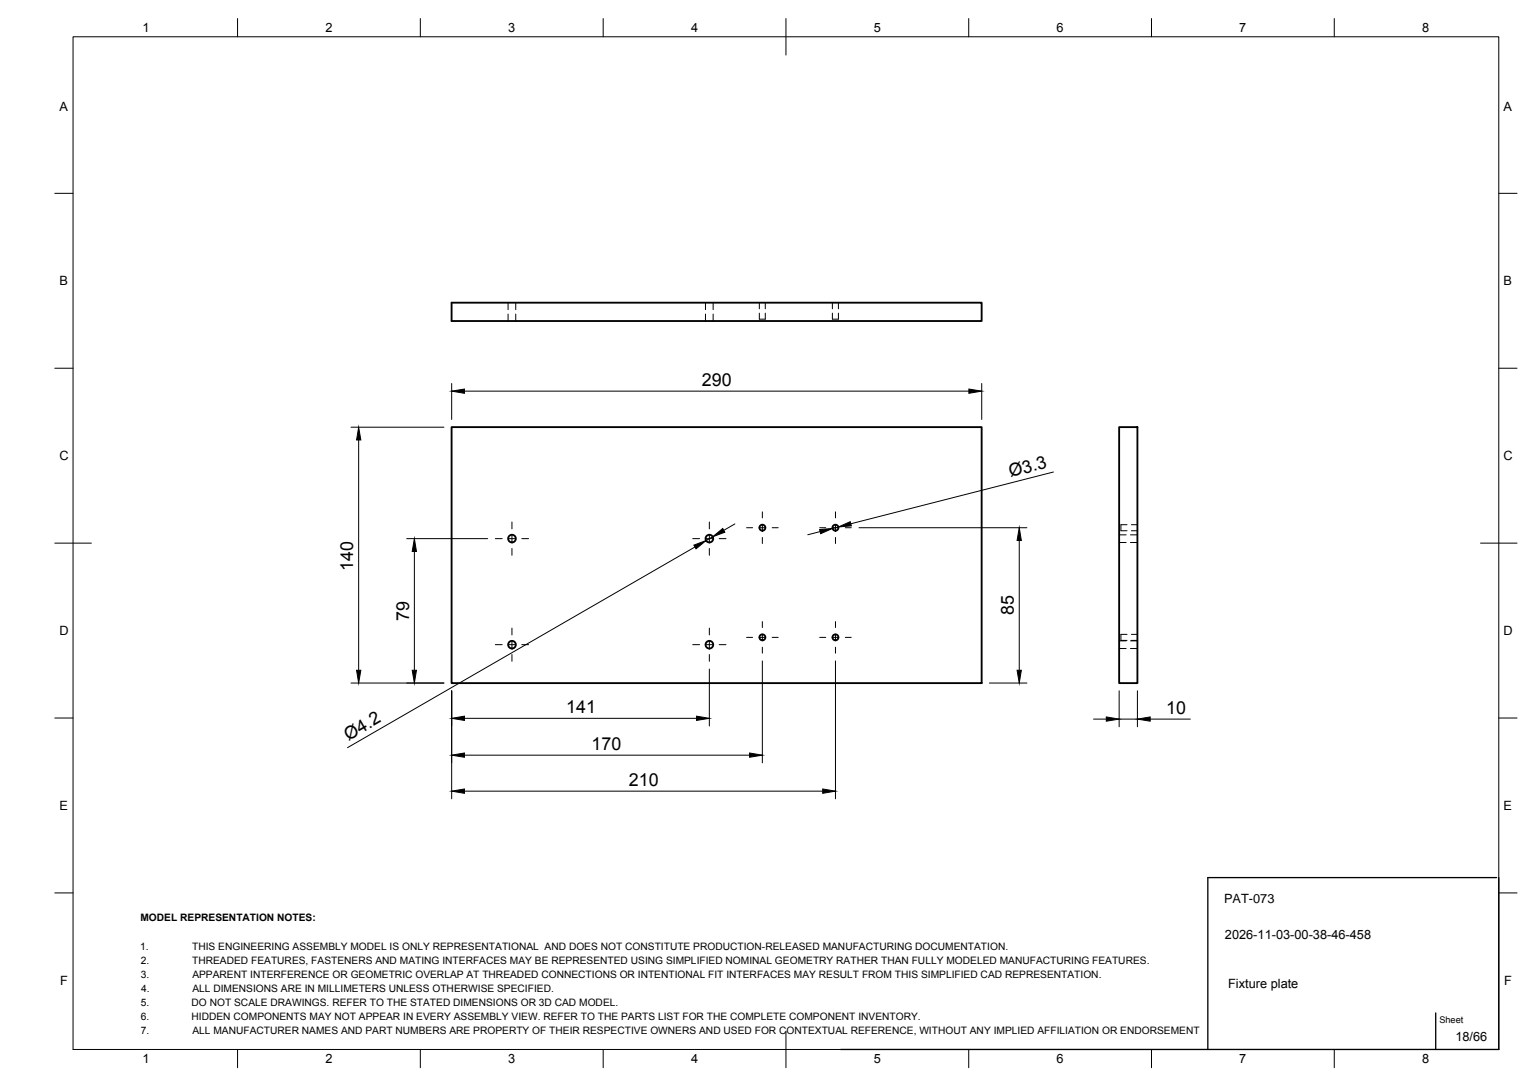
ISO-10303-21;
HEADER;
/* Generated by software containing ST-Developer
 * from STEP Tools, Inc. (www.steptools.com) 
 */

FILE_DESCRIPTION(
/* description */ ('Manual piston pump'),
/* implementation_level */ '2;1');

FILE_NAME(
/* name */ 'Fixture plate.step',
/* time_stamp */ '2026-11-02T16:54:23-08:00',
/* author */ (''),
/* organization */ (''),
/* preprocessor_version */ 'ST-DEVELOPER v20.2',
/* originating_system */ 'Autodesk Translation Framework v15.17.0.0',
/* authorisation */ '');

FILE_SCHEMA (('AUTOMOTIVE_DESIGN { 1 0 10303 214 3 1 1 }'));
ENDSEC;

DATA;
#10=MECHANICAL_DESIGN_GEOMETRIC_PRESENTATION_REPRESENTATION('',(#704),#19043);
#578=SHAPE_REPRESENTATION_RELATIONSHIP('SRR','None',#19324,#641);
#641=ADVANCED_BREP_SHAPE_REPRESENTATION('',(#775),#18991);
#704=STYLED_ITEM('',(#19661),#775);
#775=MANIFOLD_SOLID_BREP('Body1',#9489);
#889=FACE_BOUND('',#2092,.T.);
#890=FACE_BOUND('',#2093,.T.);
#891=FACE_BOUND('',#2094,.T.);
#892=FACE_BOUND('',#2095,.T.);
#893=FACE_BOUND('',#2096,.T.);
#894=FACE_BOUND('',#2097,.T.);
#895=FACE_BOUND('',#2098,.T.);
#896=FACE_BOUND('',#2099,.T.);
#897=FACE_BOUND('',#2101,.T.);
#898=FACE_BOUND('',#2102,.T.);
#899=FACE_BOUND('',#2103,.T.);
#900=FACE_BOUND('',#2104,.T.);
#1147=CYLINDRICAL_SURFACE('',#10531,0.165);
#1148=CYLINDRICAL_SURFACE('',#10535,0.165);
#1149=CYLINDRICAL_SURFACE('',#10539,0.165);
#1150=CYLINDRICAL_SURFACE('',#10543,0.165);
#1151=CYLINDRICAL_SURFACE('',#10547,0.21);
#1152=CYLINDRICAL_SURFACE('',#10550,0.21);
#1153=CYLINDRICAL_SURFACE('',#10553,0.21);
#1154=CYLINDRICAL_SURFACE('',#10556,0.21);
#1438=FACE_OUTER_BOUND('',#2075,.T.);
#1439=FACE_OUTER_BOUND('',#2076,.T.);
#1440=FACE_OUTER_BOUND('',#2077,.T.);
#1441=FACE_OUTER_BOUND('',#2078,.T.);
#1442=FACE_OUTER_BOUND('',#2079,.T.);
#1443=FACE_OUTER_BOUND('',#2080,.T.);
#1444=FACE_OUTER_BOUND('',#2081,.T.);
#1445=FACE_OUTER_BOUND('',#2082,.T.);
#1446=FACE_OUTER_BOUND('',#2083,.T.);
#1447=FACE_OUTER_BOUND('',#2084,.T.);
#1448=FACE_OUTER_BOUND('',#2085,.T.);
#1449=FACE_OUTER_BOUND('',#2086,.T.);
#1450=FACE_OUTER_BOUND('',#2087,.T.);
#1451=FACE_OUTER_BOUND('',#2088,.T.);
#1452=FACE_OUTER_BOUND('',#2089,.T.);
#1453=FACE_OUTER_BOUND('',#2090,.T.);
#1454=FACE_OUTER_BOUND('',#2091,.T.);
#1455=FACE_OUTER_BOUND('',#2100,.T.);
#2075=EDGE_LOOP('',(#6865,#6866,#6867,#6868));
#2076=EDGE_LOOP('',(#6869));
#2077=EDGE_LOOP('',(#6870,#6871,#6872,#6873));
#2078=EDGE_LOOP('',(#6874));
#2079=EDGE_LOOP('',(#6875,#6876,#6877,#6878));
#2080=EDGE_LOOP('',(#6879));
#2081=EDGE_LOOP('',(#6880,#6881,#6882,#6883));
#2082=EDGE_LOOP('',(#6884));
#2083=EDGE_LOOP('',(#6885,#6886,#6887,#6888));
#2084=EDGE_LOOP('',(#6889,#6890,#6891,#6892));
#2085=EDGE_LOOP('',(#6893,#6894,#6895,#6896));
#2086=EDGE_LOOP('',(#6897,#6898,#6899,#6900));
#2087=EDGE_LOOP('',(#6901,#6902,#6903,#6904));
#2088=EDGE_LOOP('',(#6905,#6906,#6907,#6908));
#2089=EDGE_LOOP('',(#6909,#6910,#6911,#6912));
#2090=EDGE_LOOP('',(#6913,#6914,#6915,#6916));
#2091=EDGE_LOOP('',(#6917,#6918,#6919,#6920));
#2092=EDGE_LOOP('',(#6921));
#2093=EDGE_LOOP('',(#6922));
#2094=EDGE_LOOP('',(#6923));
#2095=EDGE_LOOP('',(#6924));
#2096=EDGE_LOOP('',(#6925));
#2097=EDGE_LOOP('',(#6926));
#2098=EDGE_LOOP('',(#6927));
#2099=EDGE_LOOP('',(#6928));
#2100=EDGE_LOOP('',(#6929,#6930,#6931,#6932));
#2101=EDGE_LOOP('',(#6933));
#2102=EDGE_LOOP('',(#6934));
#2103=EDGE_LOOP('',(#6935));
#2104=EDGE_LOOP('',(#6936));
#2786=CIRCLE('',#10532,0.165);
#2787=CIRCLE('',#10533,0.165);
#2788=CIRCLE('',#10536,0.165);
#2789=CIRCLE('',#10537,0.165);
#2790=CIRCLE('',#10540,0.165);
#2791=CIRCLE('',#10541,0.165);
#2792=CIRCLE('',#10544,0.165);
#2793=CIRCLE('',#10545,0.165);
#2794=CIRCLE('',#10548,0.21);
#2795=CIRCLE('',#10549,0.21);
#2796=CIRCLE('',#10551,0.21);
#2797=CIRCLE('',#10552,0.21);
#2798=CIRCLE('',#10554,0.21);
#2799=CIRCLE('',#10555,0.21);
#2800=CIRCLE('',#10557,0.21);
#2801=CIRCLE('',#10558,0.21);
#3305=LINE('',#15337,#3909);
#3306=LINE('',#15344,#3910);
#3307=LINE('',#15351,#3911);
#3308=LINE('',#15358,#3912);
#3309=LINE('',#15365,#3913);
#3310=LINE('',#15371,#3914);
#3311=LINE('',#15377,#3915);
#3312=LINE('',#15383,#3916);
#3313=LINE('',#15388,#3917);
#3314=LINE('',#15390,#3918);
#3315=LINE('',#15392,#3919);
#3316=LINE('',#15393,#3920);
#3317=LINE('',#15396,#3921);
#3318=LINE('',#15398,#3922);
#3319=LINE('',#15399,#3923);
#3320=LINE('',#15402,#3924);
#3321=LINE('',#15404,#3925);
#3322=LINE('',#15405,#3926);
#3323=LINE('',#15407,#3927);
#3324=LINE('',#15408,#3928);
#3909=VECTOR('',#12233,0.165);
#3910=VECTOR('',#12242,0.165);
#3911=VECTOR('',#12251,0.165);
#3912=VECTOR('',#12260,0.165);
#3913=VECTOR('',#12269,0.21);
#3914=VECTOR('',#12276,0.21);
#3915=VECTOR('',#12283,0.21);
#3916=VECTOR('',#12290,0.21);
#3917=VECTOR('',#12295,1.);
#3918=VECTOR('',#12296,1.);
#3919=VECTOR('',#12297,1.);
#3920=VECTOR('',#12298,1.);
#3921=VECTOR('',#12301,1.);
#3922=VECTOR('',#12302,1.);
#3923=VECTOR('',#12303,1.);
#3924=VECTOR('',#12306,1.);
#3925=VECTOR('',#12307,1.);
#3926=VECTOR('',#12308,1.);
#3927=VECTOR('',#12311,1.);
#3928=VECTOR('',#12312,1.);
#4549=VERTEX_POINT('',#15334);
#4550=VERTEX_POINT('',#15336);
#4551=VERTEX_POINT('',#15341);
#4552=VERTEX_POINT('',#15343);
#4553=VERTEX_POINT('',#15348);
#4554=VERTEX_POINT('',#15350);
#4555=VERTEX_POINT('',#15355);
#4556=VERTEX_POINT('',#15357);
#4557=VERTEX_POINT('',#15362);
#4558=VERTEX_POINT('',#15364);
#4559=VERTEX_POINT('',#15368);
#4560=VERTEX_POINT('',#15370);
#4561=VERTEX_POINT('',#15374);
#4562=VERTEX_POINT('',#15376);
#4563=VERTEX_POINT('',#15380);
#4564=VERTEX_POINT('',#15382);
#4565=VERTEX_POINT('',#15386);
#4566=VERTEX_POINT('',#15387);
#4567=VERTEX_POINT('',#15389);
#4568=VERTEX_POINT('',#15391);
#4569=VERTEX_POINT('',#15395);
#4570=VERTEX_POINT('',#15397);
#4571=VERTEX_POINT('',#15401);
#4572=VERTEX_POINT('',#15403);
#5419=EDGE_CURVE('',#4549,#4549,#2786,.T.);
#5420=EDGE_CURVE('',#4549,#4550,#3305,.T.);
#5421=EDGE_CURVE('',#4550,#4550,#2787,.T.);
#5422=EDGE_CURVE('',#4551,#4551,#2788,.T.);
#5423=EDGE_CURVE('',#4551,#4552,#3306,.T.);
#5424=EDGE_CURVE('',#4552,#4552,#2789,.T.);
#5425=EDGE_CURVE('',#4553,#4553,#2790,.T.);
#5426=EDGE_CURVE('',#4553,#4554,#3307,.T.);
#5427=EDGE_CURVE('',#4554,#4554,#2791,.T.);
#5428=EDGE_CURVE('',#4555,#4555,#2792,.T.);
#5429=EDGE_CURVE('',#4555,#4556,#3308,.T.);
#5430=EDGE_CURVE('',#4556,#4556,#2793,.T.);
#5431=EDGE_CURVE('',#4557,#4557,#2794,.T.);
#5432=EDGE_CURVE('',#4557,#4558,#3309,.T.);
#5433=EDGE_CURVE('',#4558,#4558,#2795,.T.);
#5434=EDGE_CURVE('',#4559,#4559,#2796,.T.);
#5435=EDGE_CURVE('',#4559,#4560,#3310,.T.);
#5436=EDGE_CURVE('',#4560,#4560,#2797,.T.);
#5437=EDGE_CURVE('',#4561,#4561,#2798,.T.);
#5438=EDGE_CURVE('',#4561,#4562,#3311,.T.);
#5439=EDGE_CURVE('',#4562,#4562,#2799,.T.);
#5440=EDGE_CURVE('',#4563,#4563,#2800,.T.);
#5441=EDGE_CURVE('',#4563,#4564,#3312,.T.);
#5442=EDGE_CURVE('',#4564,#4564,#2801,.T.);
#5443=EDGE_CURVE('',#4565,#4566,#3313,.T.);
#5444=EDGE_CURVE('',#4566,#4567,#3314,.T.);
#5445=EDGE_CURVE('',#4568,#4567,#3315,.T.);
#5446=EDGE_CURVE('',#4565,#4568,#3316,.T.);
#5447=EDGE_CURVE('',#4569,#4565,#3317,.T.);
#5448=EDGE_CURVE('',#4570,#4568,#3318,.T.);
#5449=EDGE_CURVE('',#4569,#4570,#3319,.T.);
#5450=EDGE_CURVE('',#4571,#4569,#3320,.T.);
#5451=EDGE_CURVE('',#4572,#4570,#3321,.T.);
#5452=EDGE_CURVE('',#4571,#4572,#3322,.T.);
#5453=EDGE_CURVE('',#4566,#4571,#3323,.T.);
#5454=EDGE_CURVE('',#4567,#4572,#3324,.T.);
#6865=ORIENTED_EDGE('',*,*,#5419,.F.);
#6866=ORIENTED_EDGE('',*,*,#5420,.T.);
#6867=ORIENTED_EDGE('',*,*,#5421,.F.);
#6868=ORIENTED_EDGE('',*,*,#5420,.F.);
#6869=ORIENTED_EDGE('',*,*,#5419,.T.);
#6870=ORIENTED_EDGE('',*,*,#5422,.F.);
#6871=ORIENTED_EDGE('',*,*,#5423,.T.);
#6872=ORIENTED_EDGE('',*,*,#5424,.F.);
#6873=ORIENTED_EDGE('',*,*,#5423,.F.);
#6874=ORIENTED_EDGE('',*,*,#5422,.T.);
#6875=ORIENTED_EDGE('',*,*,#5425,.F.);
#6876=ORIENTED_EDGE('',*,*,#5426,.T.);
#6877=ORIENTED_EDGE('',*,*,#5427,.F.);
#6878=ORIENTED_EDGE('',*,*,#5426,.F.);
#6879=ORIENTED_EDGE('',*,*,#5425,.T.);
#6880=ORIENTED_EDGE('',*,*,#5428,.F.);
#6881=ORIENTED_EDGE('',*,*,#5429,.T.);
#6882=ORIENTED_EDGE('',*,*,#5430,.F.);
#6883=ORIENTED_EDGE('',*,*,#5429,.F.);
#6884=ORIENTED_EDGE('',*,*,#5428,.T.);
#6885=ORIENTED_EDGE('',*,*,#5431,.F.);
#6886=ORIENTED_EDGE('',*,*,#5432,.T.);
#6887=ORIENTED_EDGE('',*,*,#5433,.F.);
#6888=ORIENTED_EDGE('',*,*,#5432,.F.);
#6889=ORIENTED_EDGE('',*,*,#5434,.F.);
#6890=ORIENTED_EDGE('',*,*,#5435,.T.);
#6891=ORIENTED_EDGE('',*,*,#5436,.F.);
#6892=ORIENTED_EDGE('',*,*,#5435,.F.);
#6893=ORIENTED_EDGE('',*,*,#5437,.F.);
#6894=ORIENTED_EDGE('',*,*,#5438,.T.);
#6895=ORIENTED_EDGE('',*,*,#5439,.F.);
#6896=ORIENTED_EDGE('',*,*,#5438,.F.);
#6897=ORIENTED_EDGE('',*,*,#5440,.F.);
#6898=ORIENTED_EDGE('',*,*,#5441,.T.);
#6899=ORIENTED_EDGE('',*,*,#5442,.F.);
#6900=ORIENTED_EDGE('',*,*,#5441,.F.);
#6901=ORIENTED_EDGE('',*,*,#5443,.T.);
#6902=ORIENTED_EDGE('',*,*,#5444,.T.);
#6903=ORIENTED_EDGE('',*,*,#5445,.F.);
#6904=ORIENTED_EDGE('',*,*,#5446,.F.);
#6905=ORIENTED_EDGE('',*,*,#5447,.T.);
#6906=ORIENTED_EDGE('',*,*,#5446,.T.);
#6907=ORIENTED_EDGE('',*,*,#5448,.F.);
#6908=ORIENTED_EDGE('',*,*,#5449,.F.);
#6909=ORIENTED_EDGE('',*,*,#5450,.T.);
#6910=ORIENTED_EDGE('',*,*,#5449,.T.);
#6911=ORIENTED_EDGE('',*,*,#5451,.F.);
#6912=ORIENTED_EDGE('',*,*,#5452,.F.);
#6913=ORIENTED_EDGE('',*,*,#5453,.T.);
#6914=ORIENTED_EDGE('',*,*,#5452,.T.);
#6915=ORIENTED_EDGE('',*,*,#5454,.F.);
#6916=ORIENTED_EDGE('',*,*,#5444,.F.);
#6917=ORIENTED_EDGE('',*,*,#5454,.T.);
#6918=ORIENTED_EDGE('',*,*,#5451,.T.);
#6919=ORIENTED_EDGE('',*,*,#5448,.T.);
#6920=ORIENTED_EDGE('',*,*,#5445,.T.);
#6921=ORIENTED_EDGE('',*,*,#5442,.T.);
#6922=ORIENTED_EDGE('',*,*,#5439,.T.);
#6923=ORIENTED_EDGE('',*,*,#5436,.T.);
#6924=ORIENTED_EDGE('',*,*,#5433,.T.);
#6925=ORIENTED_EDGE('',*,*,#5430,.T.);
#6926=ORIENTED_EDGE('',*,*,#5427,.T.);
#6927=ORIENTED_EDGE('',*,*,#5424,.T.);
#6928=ORIENTED_EDGE('',*,*,#5421,.T.);
#6929=ORIENTED_EDGE('',*,*,#5453,.F.);
#6930=ORIENTED_EDGE('',*,*,#5443,.F.);
#6931=ORIENTED_EDGE('',*,*,#5447,.F.);
#6932=ORIENTED_EDGE('',*,*,#5450,.F.);
#6933=ORIENTED_EDGE('',*,*,#5431,.T.);
#6934=ORIENTED_EDGE('',*,*,#5434,.T.);
#6935=ORIENTED_EDGE('',*,*,#5437,.T.);
#6936=ORIENTED_EDGE('',*,*,#5440,.T.);
#8655=PLANE('',#10534);
#8656=PLANE('',#10538);
#8657=PLANE('',#10542);
#8658=PLANE('',#10546);
#8659=PLANE('',#10559);
#8660=PLANE('',#10560);
#8661=PLANE('',#10561);
#8662=PLANE('',#10562);
#8663=PLANE('',#10563);
#8664=PLANE('',#10564);
#9043=ADVANCED_FACE('',(#1438),#1147,.F.);
#9044=ADVANCED_FACE('',(#1439),#8655,.T.);
#9045=ADVANCED_FACE('',(#1440),#1148,.F.);
#9046=ADVANCED_FACE('',(#1441),#8656,.T.);
#9047=ADVANCED_FACE('',(#1442),#1149,.F.);
#9048=ADVANCED_FACE('',(#1443),#8657,.T.);
#9049=ADVANCED_FACE('',(#1444),#1150,.F.);
#9050=ADVANCED_FACE('',(#1445),#8658,.T.);
#9051=ADVANCED_FACE('',(#1446),#1151,.F.);
#9052=ADVANCED_FACE('',(#1447),#1152,.F.);
#9053=ADVANCED_FACE('',(#1448),#1153,.F.);
#9054=ADVANCED_FACE('',(#1449),#1154,.F.);
#9055=ADVANCED_FACE('',(#1450),#8659,.T.);
#9056=ADVANCED_FACE('',(#1451),#8660,.T.);
#9057=ADVANCED_FACE('',(#1452),#8661,.T.);
#9058=ADVANCED_FACE('',(#1453),#8662,.T.);
#9059=ADVANCED_FACE('',(#1454,#889,#890,#891,#892,#893,#894,#895,#896),
#8663,.T.);
#9060=ADVANCED_FACE('',(#1455,#897,#898,#899,#900),#8664,.F.);
#9489=CLOSED_SHELL('',(#9043,#9044,#9045,#9046,#9047,#9048,#9049,#9050,
#9051,#9052,#9053,#9054,#9055,#9056,#9057,#9058,#9059,#9060));
#10530=AXIS2_PLACEMENT_3D('',#15332,#12227,#12228);
#10531=AXIS2_PLACEMENT_3D('',#15333,#12229,#12230);
#10532=AXIS2_PLACEMENT_3D('',#15335,#12231,#12232);
#10533=AXIS2_PLACEMENT_3D('',#15338,#12234,#12235);
#10534=AXIS2_PLACEMENT_3D('',#15339,#12236,#12237);
#10535=AXIS2_PLACEMENT_3D('',#15340,#12238,#12239);
#10536=AXIS2_PLACEMENT_3D('',#15342,#12240,#12241);
#10537=AXIS2_PLACEMENT_3D('',#15345,#12243,#12244);
#10538=AXIS2_PLACEMENT_3D('',#15346,#12245,#12246);
#10539=AXIS2_PLACEMENT_3D('',#15347,#12247,#12248);
#10540=AXIS2_PLACEMENT_3D('',#15349,#12249,#12250);
#10541=AXIS2_PLACEMENT_3D('',#15352,#12252,#12253);
#10542=AXIS2_PLACEMENT_3D('',#15353,#12254,#12255);
#10543=AXIS2_PLACEMENT_3D('',#15354,#12256,#12257);
#10544=AXIS2_PLACEMENT_3D('',#15356,#12258,#12259);
#10545=AXIS2_PLACEMENT_3D('',#15359,#12261,#12262);
#10546=AXIS2_PLACEMENT_3D('',#15360,#12263,#12264);
#10547=AXIS2_PLACEMENT_3D('',#15361,#12265,#12266);
#10548=AXIS2_PLACEMENT_3D('',#15363,#12267,#12268);
#10549=AXIS2_PLACEMENT_3D('',#15366,#12270,#12271);
#10550=AXIS2_PLACEMENT_3D('',#15367,#12272,#12273);
#10551=AXIS2_PLACEMENT_3D('',#15369,#12274,#12275);
#10552=AXIS2_PLACEMENT_3D('',#15372,#12277,#12278);
#10553=AXIS2_PLACEMENT_3D('',#15373,#12279,#12280);
#10554=AXIS2_PLACEMENT_3D('',#15375,#12281,#12282);
#10555=AXIS2_PLACEMENT_3D('',#15378,#12284,#12285);
#10556=AXIS2_PLACEMENT_3D('',#15379,#12286,#12287);
#10557=AXIS2_PLACEMENT_3D('',#15381,#12288,#12289);
#10558=AXIS2_PLACEMENT_3D('',#15384,#12291,#12292);
#10559=AXIS2_PLACEMENT_3D('',#15385,#12293,#12294);
#10560=AXIS2_PLACEMENT_3D('',#15394,#12299,#12300);
#10561=AXIS2_PLACEMENT_3D('',#15400,#12304,#12305);
#10562=AXIS2_PLACEMENT_3D('',#15406,#12309,#12310);
#10563=AXIS2_PLACEMENT_3D('',#15409,#12313,#12314);
#10564=AXIS2_PLACEMENT_3D('',#15410,#12315,#12316);
#12227=DIRECTION('axis',(0.,0.,1.));
#12228=DIRECTION('refdir',(1.,0.,0.));
#12229=DIRECTION('center_axis',(0.,0.,1.));
#12230=DIRECTION('ref_axis',(1.,0.,0.));
#12231=DIRECTION('center_axis',(0.,0.,1.));
#12232=DIRECTION('ref_axis',(1.,0.,0.));
#12233=DIRECTION('',(0.,0.,1.));
#12234=DIRECTION('center_axis',(0.,0.,-1.));
#12235=DIRECTION('ref_axis',(1.,0.,0.));
#12236=DIRECTION('center_axis',(0.,0.,1.));
#12237=DIRECTION('ref_axis',(1.,0.,0.));
#12238=DIRECTION('center_axis',(0.,0.,1.));
#12239=DIRECTION('ref_axis',(1.,0.,0.));
#12240=DIRECTION('center_axis',(0.,0.,1.));
#12241=DIRECTION('ref_axis',(1.,0.,0.));
#12242=DIRECTION('',(0.,0.,1.));
#12243=DIRECTION('center_axis',(0.,0.,-1.));
#12244=DIRECTION('ref_axis',(1.,0.,0.));
#12245=DIRECTION('center_axis',(0.,0.,1.));
#12246=DIRECTION('ref_axis',(1.,0.,0.));
#12247=DIRECTION('center_axis',(0.,0.,1.));
#12248=DIRECTION('ref_axis',(1.,0.,0.));
#12249=DIRECTION('center_axis',(0.,0.,1.));
#12250=DIRECTION('ref_axis',(1.,0.,0.));
#12251=DIRECTION('',(0.,0.,1.));
#12252=DIRECTION('center_axis',(0.,0.,-1.));
#12253=DIRECTION('ref_axis',(1.,0.,0.));
#12254=DIRECTION('center_axis',(0.,0.,1.));
#12255=DIRECTION('ref_axis',(1.,0.,0.));
#12256=DIRECTION('center_axis',(0.,0.,1.));
#12257=DIRECTION('ref_axis',(1.,0.,0.));
#12258=DIRECTION('center_axis',(0.,0.,1.));
#12259=DIRECTION('ref_axis',(1.,0.,0.));
#12260=DIRECTION('',(0.,0.,1.));
#12261=DIRECTION('center_axis',(0.,0.,-1.));
#12262=DIRECTION('ref_axis',(1.,0.,0.));
#12263=DIRECTION('center_axis',(0.,0.,1.));
#12264=DIRECTION('ref_axis',(1.,0.,0.));
#12265=DIRECTION('center_axis',(0.,0.,1.));
#12266=DIRECTION('ref_axis',(1.,0.,0.));
#12267=DIRECTION('center_axis',(0.,0.,1.));
#12268=DIRECTION('ref_axis',(1.,0.,0.));
#12269=DIRECTION('',(0.,0.,1.));
#12270=DIRECTION('center_axis',(0.,0.,-1.));
#12271=DIRECTION('ref_axis',(1.,0.,0.));
#12272=DIRECTION('center_axis',(0.,0.,1.));
#12273=DIRECTION('ref_axis',(1.,0.,0.));
#12274=DIRECTION('center_axis',(0.,0.,1.));
#12275=DIRECTION('ref_axis',(1.,0.,0.));
#12276=DIRECTION('',(0.,0.,1.));
#12277=DIRECTION('center_axis',(0.,0.,-1.));
#12278=DIRECTION('ref_axis',(1.,0.,0.));
#12279=DIRECTION('center_axis',(0.,0.,1.));
#12280=DIRECTION('ref_axis',(1.,0.,0.));
#12281=DIRECTION('center_axis',(0.,0.,1.));
#12282=DIRECTION('ref_axis',(1.,0.,0.));
#12283=DIRECTION('',(0.,0.,1.));
#12284=DIRECTION('center_axis',(0.,0.,-1.));
#12285=DIRECTION('ref_axis',(1.,0.,0.));
#12286=DIRECTION('center_axis',(0.,0.,1.));
#12287=DIRECTION('ref_axis',(1.,0.,0.));
#12288=DIRECTION('center_axis',(0.,0.,1.));
#12289=DIRECTION('ref_axis',(1.,0.,0.));
#12290=DIRECTION('',(0.,0.,1.));
#12291=DIRECTION('center_axis',(0.,0.,-1.));
#12292=DIRECTION('ref_axis',(1.,0.,0.));
#12293=DIRECTION('center_axis',(0.,1.,0.));
#12294=DIRECTION('ref_axis',(-1.,0.,0.));
#12295=DIRECTION('',(-1.,0.,0.));
#12296=DIRECTION('',(0.,0.,1.));
#12297=DIRECTION('',(-1.,0.,0.));
#12298=DIRECTION('',(0.,0.,1.));
#12299=DIRECTION('center_axis',(1.,0.,0.));
#12300=DIRECTION('ref_axis',(0.,1.,0.));
#12301=DIRECTION('',(0.,1.,0.));
#12302=DIRECTION('',(0.,1.,0.));
#12303=DIRECTION('',(0.,0.,1.));
#12304=DIRECTION('center_axis',(0.,-1.,0.));
#12305=DIRECTION('ref_axis',(1.,0.,0.));
#12306=DIRECTION('',(1.,0.,0.));
#12307=DIRECTION('',(1.,0.,0.));
#12308=DIRECTION('',(0.,0.,1.));
#12309=DIRECTION('center_axis',(-1.,0.,0.));
#12310=DIRECTION('ref_axis',(0.,-1.,0.));
#12311=DIRECTION('',(0.,-1.,0.));
#12312=DIRECTION('',(0.,-1.,0.));
#12313=DIRECTION('center_axis',(0.,0.,1.));
#12314=DIRECTION('ref_axis',(1.,0.,0.));
#12315=DIRECTION('center_axis',(0.,0.,1.));
#12316=DIRECTION('ref_axis',(1.,0.,0.));
#15332=CARTESIAN_POINT('',(0.,0.,0.));
#15333=CARTESIAN_POINT('Origin',(3.5,-2.,-0.9));
#15334=CARTESIAN_POINT('',(3.335,-2.,-0.9));
#15335=CARTESIAN_POINT('Origin',(3.5,-2.,-0.9));
#15336=CARTESIAN_POINT('',(3.335,-2.,0.));
#15337=CARTESIAN_POINT('',(3.335,-2.,-0.9));
#15338=CARTESIAN_POINT('Origin',(3.5,-2.,0.));
#15339=CARTESIAN_POINT('Origin',(3.5,-2.,-0.9));
#15340=CARTESIAN_POINT('Origin',(3.5,-6.,-0.9));
#15341=CARTESIAN_POINT('',(3.335,-6.,-0.9));
#15342=CARTESIAN_POINT('Origin',(3.5,-6.,-0.9));
#15343=CARTESIAN_POINT('',(3.335,-6.,0.));
#15344=CARTESIAN_POINT('',(3.335,-6.,-0.9));
#15345=CARTESIAN_POINT('Origin',(3.5,-6.,0.));
#15346=CARTESIAN_POINT('Origin',(3.5,-6.,-0.9));
#15347=CARTESIAN_POINT('Origin',(-2.5,-2.,-0.9));
#15348=CARTESIAN_POINT('',(-2.665,-2.,-0.9));
#15349=CARTESIAN_POINT('Origin',(-2.5,-2.,-0.9));
#15350=CARTESIAN_POINT('',(-2.665,-2.,0.));
#15351=CARTESIAN_POINT('',(-2.665,-2.,-0.9));
#15352=CARTESIAN_POINT('Origin',(-2.5,-2.,0.));
#15353=CARTESIAN_POINT('Origin',(-2.5,-2.,-0.9));
#15354=CARTESIAN_POINT('Origin',(-2.5,-6.,-0.9));
#15355=CARTESIAN_POINT('',(-2.665,-6.,-0.9));
#15356=CARTESIAN_POINT('Origin',(-2.5,-6.,-0.9));
#15357=CARTESIAN_POINT('',(-2.665,-6.,0.));
#15358=CARTESIAN_POINT('',(-2.665,-6.,-0.9));
#15359=CARTESIAN_POINT('Origin',(-2.5,-6.,0.));
#15360=CARTESIAN_POINT('Origin',(-2.5,-6.,-0.9));
#15361=CARTESIAN_POINT('Origin',(2.9,11.7,-1.1));
#15362=CARTESIAN_POINT('',(2.69,11.7,-1.));
#15363=CARTESIAN_POINT('Origin',(2.9,11.7,-1.));
#15364=CARTESIAN_POINT('',(2.69,11.7,0.));
#15365=CARTESIAN_POINT('',(2.69,11.7,-1.1));
#15366=CARTESIAN_POINT('Origin',(2.9,11.7,0.));
#15367=CARTESIAN_POINT('Origin',(2.9,0.9,-1.1));
#15368=CARTESIAN_POINT('',(2.69,0.9,-1.));
#15369=CARTESIAN_POINT('Origin',(2.9,0.9,-1.));
#15370=CARTESIAN_POINT('',(2.69,0.9,0.));
#15371=CARTESIAN_POINT('',(2.69,0.9,-1.1));
#15372=CARTESIAN_POINT('Origin',(2.9,0.9,0.));
#15373=CARTESIAN_POINT('Origin',(-2.9,11.7,-1.1));
#15374=CARTESIAN_POINT('',(-3.11,11.7,-1.));
#15375=CARTESIAN_POINT('Origin',(-2.9,11.7,-1.));
#15376=CARTESIAN_POINT('',(-3.11,11.7,0.));
#15377=CARTESIAN_POINT('',(-3.11,11.7,-1.1));
#15378=CARTESIAN_POINT('Origin',(-2.9,11.7,0.));
#15379=CARTESIAN_POINT('Origin',(-2.9,0.9,-1.1));
#15380=CARTESIAN_POINT('',(-3.11,0.9,-1.));
#15381=CARTESIAN_POINT('Origin',(-2.9,0.9,-1.));
#15382=CARTESIAN_POINT('',(-3.11,0.9,0.));
#15383=CARTESIAN_POINT('',(-3.11,0.9,-1.1));
#15384=CARTESIAN_POINT('Origin',(-2.9,0.9,0.));
#15385=CARTESIAN_POINT('Origin',(9.,15.,-1.));
#15386=CARTESIAN_POINT('',(9.,15.,-1.));
#15387=CARTESIAN_POINT('',(-5.,15.,-1.));
#15388=CARTESIAN_POINT('',(9.,15.,-1.));
#15389=CARTESIAN_POINT('',(-5.,15.,0.));
#15390=CARTESIAN_POINT('',(-5.,15.,-1.));
#15391=CARTESIAN_POINT('',(9.,15.,0.));
#15392=CARTESIAN_POINT('',(9.,15.,0.));
#15393=CARTESIAN_POINT('',(9.,15.,-1.));
#15394=CARTESIAN_POINT('Origin',(9.,-14.,-1.));
#15395=CARTESIAN_POINT('',(9.,-14.,-1.));
#15396=CARTESIAN_POINT('',(9.,-14.,-1.));
#15397=CARTESIAN_POINT('',(9.,-14.,0.));
#15398=CARTESIAN_POINT('',(9.,-14.,0.));
#15399=CARTESIAN_POINT('',(9.,-14.,-1.));
#15400=CARTESIAN_POINT('Origin',(-5.,-14.,-1.));
#15401=CARTESIAN_POINT('',(-5.,-14.,-1.));
#15402=CARTESIAN_POINT('',(-5.,-14.,-1.));
#15403=CARTESIAN_POINT('',(-5.,-14.,0.));
#15404=CARTESIAN_POINT('',(-5.,-14.,0.));
#15405=CARTESIAN_POINT('',(-5.,-14.,-1.));
#15406=CARTESIAN_POINT('Origin',(-5.,15.,-1.));
#15407=CARTESIAN_POINT('',(-5.,15.,-1.));
#15408=CARTESIAN_POINT('',(-5.,15.,0.));
#15409=CARTESIAN_POINT('Origin',(2.,0.5,0.));
#15410=CARTESIAN_POINT('Origin',(2.,0.5,-1.));
#18920=UNCERTAINTY_MEASURE_WITH_UNIT(LENGTH_MEASURE(0.001),#19044,
'DISTANCE_ACCURACY_VALUE',
'Maximum model space distance between geometric entities at asserted c
onnectivities');
#18972=UNCERTAINTY_MEASURE_WITH_UNIT(LENGTH_MEASURE(0.001),#19044,
'DISTANCE_ACCURACY_VALUE',
'Maximum model space distance between geometric entities at asserted c
onnectivities');
#18991=(
GEOMETRIC_REPRESENTATION_CONTEXT(3)
GLOBAL_UNCERTAINTY_ASSIGNED_CONTEXT((#18920))
GLOBAL_UNIT_ASSIGNED_CONTEXT((#19044,#19046,#19047))
REPRESENTATION_CONTEXT('','3D')
);
#19043=(
GEOMETRIC_REPRESENTATION_CONTEXT(3)
GLOBAL_UNCERTAINTY_ASSIGNED_CONTEXT((#18972))
GLOBAL_UNIT_ASSIGNED_CONTEXT((#19044,#19046,#19047))
REPRESENTATION_CONTEXT('','3D')
);
#19044=(
LENGTH_UNIT()
NAMED_UNIT(*)
SI_UNIT(.CENTI.,.METRE.)
);
#19046=(
NAMED_UNIT(*)
PLANE_ANGLE_UNIT()
SI_UNIT($,.RADIAN.)
);
#19047=(
NAMED_UNIT(*)
SI_UNIT($,.STERADIAN.)
SOLID_ANGLE_UNIT()
);
#19066=SHAPE_DEFINITION_REPRESENTATION(#19136,#19324);
#19136=PRODUCT_DEFINITION_SHAPE('',$,#19395);
#19324=SHAPE_REPRESENTATION('',(#10530),#18991);
#19376=PRODUCT_DEFINITION_CONTEXT('part definition',#19588,'design');
#19395=PRODUCT_DEFINITION('2026-11-03-00-38-46-458','Fixture plate',#19465,
#19376);
#19465=PRODUCT_DEFINITION_FORMATION('',$,#19608);
#19588=APPLICATION_CONTEXT(
'Core Data for Automotive Mechanical Design Process');
#19589=PRODUCT_CONTEXT('part definition',#19588,'mechanical');
#19608=PRODUCT('2026-11-03-00-38-46-458','Fixture plate',
'Fixture plate',(#19589));
#19661=PRESENTATION_STYLE_ASSIGNMENT((#19667));
#19667=SURFACE_STYLE_USAGE(.BOTH.,#19673);
#19673=SURFACE_SIDE_STYLE('',(#19679));
#19679=SURFACE_STYLE_FILL_AREA(#19685);
#19685=FILL_AREA_STYLE('CAD Library Painted - Engineering blue',(#19691));
#19691=FILL_AREA_STYLE_COLOUR('CAD Library Painted - Engineering blue',
#19697);
#19697=COLOUR_RGB('CAD Library Painted - Engineering blue',0.12156862745098,
0.356862745098039,0.6);
ENDSEC;
END-ISO-10303-21;
